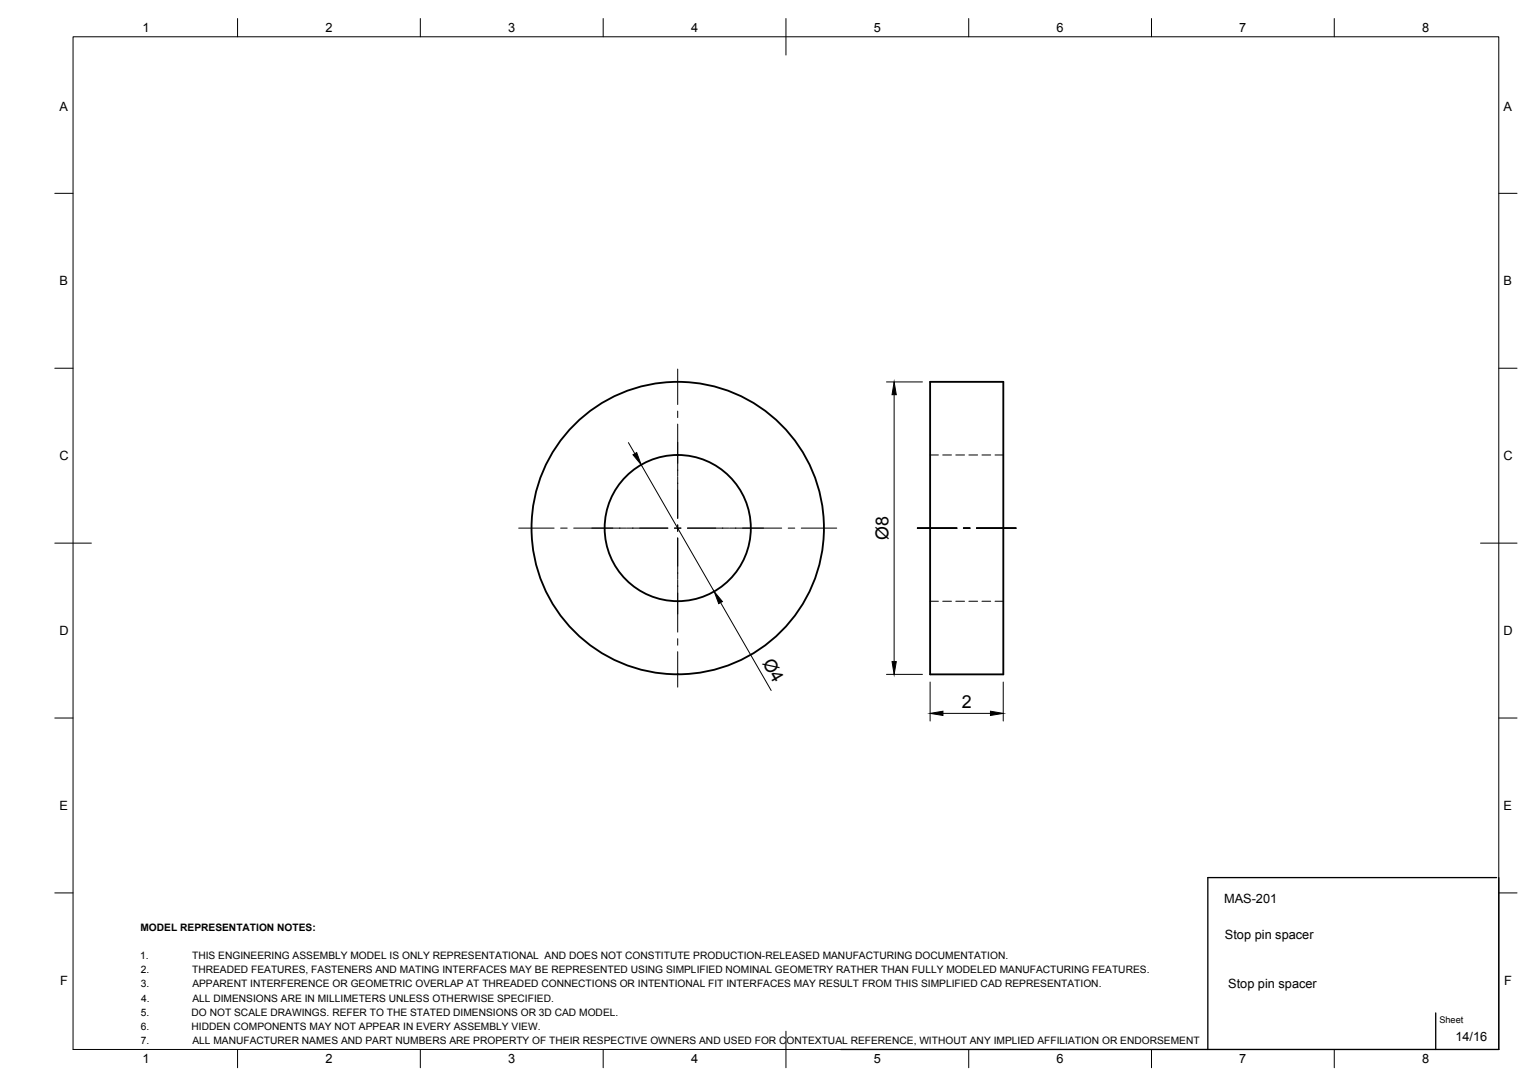
ISO-10303-21;
HEADER;
/* Generated by software containing ST-Developer
 * from STEP Tools, Inc. (www.steptools.com) 
 */

FILE_DESCRIPTION(
/* description */ ('Independent manual two-gate roller-track escapement for nominal30mm d
iameter20mm wide feed rollers. Opposed gates are driven by native capt
ured pin-slot loops with positive curved-slot travel stops at\X\B116de
g. Repeated gate/pin/washer/clip instances, adapted native common bear
ing families, full retaining lips and rotating polymer grip. External 
workpieces, gravity feeder/incline and mount anchors outside assembly.
 No powered-feed compatibility, impact, capacity, safety, force, wear 
or life rating.'),
/* implementation_level */ '2;1');

FILE_NAME(
/* name */ 'Stop pin spacer.step',
/* time_stamp */ '2026-11-08T18:43:23-08:00',
/* author */ (''),
/* organization */ (''),
/* preprocessor_version */ 'ST-DEVELOPER v20.2',
/* originating_system */ 'Autodesk Translation Framework v15.17.0.0',
/* authorisation */ '');

FILE_SCHEMA (('AUTOMOTIVE_DESIGN { 1 0 10303 214 3 1 1 }'));
ENDSEC;

DATA;
#10=MECHANICAL_DESIGN_GEOMETRIC_PRESENTATION_REPRESENTATION('',(#468),#19863);
#430=SHAPE_REPRESENTATION_RELATIONSHIP('SRR','None',#19948,#449);
#449=ADVANCED_BREP_SHAPE_REPRESENTATION('',(#487),#19857);
#468=STYLED_ITEM('',(#20043),#487);
#487=MANIFOLD_SOLID_BREP('Body1',#6437);
#862=LINE('',#15977,#1327);
#863=LINE('',#15983,#1328);
#1327=VECTOR('',#8336,2.);
#1328=VECTOR('',#8343,4.);
#1560=CYLINDRICAL_SURFACE('',#7039,2.);
#1561=CYLINDRICAL_SURFACE('',#7042,4.);
#1676=FACE_BOUND('',#2373,.T.);
#1677=FACE_BOUND('',#2375,.T.);
#1952=FACE_OUTER_BOUND('',#2370,.T.);
#1953=FACE_OUTER_BOUND('',#2371,.T.);
#1954=FACE_OUTER_BOUND('',#2372,.T.);
#1955=FACE_OUTER_BOUND('',#2374,.T.);
#2370=EDGE_LOOP('',(#5457,#5458,#5459,#5460));
#2371=EDGE_LOOP('',(#5461,#5462,#5463,#5464));
#2372=EDGE_LOOP('',(#5465));
#2373=EDGE_LOOP('',(#5466));
#2374=EDGE_LOOP('',(#5467));
#2375=EDGE_LOOP('',(#5468));
#2586=CIRCLE('',#7040,2.);
#2587=CIRCLE('',#7041,2.);
#2588=CIRCLE('',#7043,4.);
#2589=CIRCLE('',#7044,4.);
#3064=VERTEX_POINT('',#15974);
#3065=VERTEX_POINT('',#15976);
#3066=VERTEX_POINT('',#15980);
#3067=VERTEX_POINT('',#15982);
#3887=EDGE_CURVE('',#3064,#3064,#2586,.T.);
#3888=EDGE_CURVE('',#3064,#3065,#862,.T.);
#3889=EDGE_CURVE('',#3065,#3065,#2587,.T.);
#3890=EDGE_CURVE('',#3066,#3066,#2588,.T.);
#3891=EDGE_CURVE('',#3066,#3067,#863,.T.);
#3892=EDGE_CURVE('',#3067,#3067,#2589,.T.);
#5457=ORIENTED_EDGE('',*,*,#3887,.F.);
#5458=ORIENTED_EDGE('',*,*,#3888,.T.);
#5459=ORIENTED_EDGE('',*,*,#3889,.T.);
#5460=ORIENTED_EDGE('',*,*,#3888,.F.);
#5461=ORIENTED_EDGE('',*,*,#3890,.F.);
#5462=ORIENTED_EDGE('',*,*,#3891,.T.);
#5463=ORIENTED_EDGE('',*,*,#3892,.T.);
#5464=ORIENTED_EDGE('',*,*,#3891,.F.);
#5465=ORIENTED_EDGE('',*,*,#3890,.T.);
#5466=ORIENTED_EDGE('',*,*,#3887,.T.);
#5467=ORIENTED_EDGE('',*,*,#3892,.F.);
#5468=ORIENTED_EDGE('',*,*,#3889,.F.);
#6035=PLANE('',#7045);
#6036=PLANE('',#7046);
#6331=ADVANCED_FACE('',(#1952),#1560,.F.);
#6332=ADVANCED_FACE('',(#1953),#1561,.T.);
#6333=ADVANCED_FACE('',(#1954,#1676),#6035,.T.);
#6334=ADVANCED_FACE('',(#1955,#1677),#6036,.F.);
#6437=CLOSED_SHELL('',(#6331,#6332,#6333,#6334));
#7038=AXIS2_PLACEMENT_3D('',#15972,#8330,#8331);
#7039=AXIS2_PLACEMENT_3D('',#15973,#8332,#8333);
#7040=AXIS2_PLACEMENT_3D('',#15975,#8334,#8335);
#7041=AXIS2_PLACEMENT_3D('',#15978,#8337,#8338);
#7042=AXIS2_PLACEMENT_3D('',#15979,#8339,#8340);
#7043=AXIS2_PLACEMENT_3D('',#15981,#8341,#8342);
#7044=AXIS2_PLACEMENT_3D('',#15984,#8344,#8345);
#7045=AXIS2_PLACEMENT_3D('',#15985,#8346,#8347);
#7046=AXIS2_PLACEMENT_3D('',#15986,#8348,#8349);
#8330=DIRECTION('axis',(0.,0.,1.));
#8331=DIRECTION('refdir',(1.,0.,0.));
#8332=DIRECTION('center_axis',(0.,0.,1.));
#8333=DIRECTION('ref_axis',(1.,0.,0.));
#8334=DIRECTION('center_axis',(0.,0.,-1.));
#8335=DIRECTION('ref_axis',(1.,0.,0.));
#8336=DIRECTION('',(0.,0.,-1.));
#8337=DIRECTION('center_axis',(0.,0.,-1.));
#8338=DIRECTION('ref_axis',(1.,0.,0.));
#8339=DIRECTION('center_axis',(0.,0.,1.));
#8340=DIRECTION('ref_axis',(1.,0.,0.));
#8341=DIRECTION('center_axis',(0.,0.,1.));
#8342=DIRECTION('ref_axis',(1.,0.,0.));
#8343=DIRECTION('',(0.,0.,-1.));
#8344=DIRECTION('center_axis',(0.,0.,1.));
#8345=DIRECTION('ref_axis',(1.,0.,0.));
#8346=DIRECTION('center_axis',(0.,0.,1.));
#8347=DIRECTION('ref_axis',(1.,0.,0.));
#8348=DIRECTION('center_axis',(0.,0.,1.));
#8349=DIRECTION('ref_axis',(1.,0.,0.));
#15972=CARTESIAN_POINT('',(0.,0.,0.));
#15973=CARTESIAN_POINT('Origin',(0.,0.,0.));
#15974=CARTESIAN_POINT('',(-2.,-2.44929359829471E-16,2.));
#15975=CARTESIAN_POINT('Origin',(0.,0.,2.));
#15976=CARTESIAN_POINT('',(-2.,-2.44929359829471E-16,0.));
#15977=CARTESIAN_POINT('',(-2.,-2.44929359829471E-16,0.));
#15978=CARTESIAN_POINT('Origin',(0.,0.,0.));
#15979=CARTESIAN_POINT('Origin',(0.,0.,0.));
#15980=CARTESIAN_POINT('',(-4.,-4.89858719658941E-16,2.));
#15981=CARTESIAN_POINT('Origin',(0.,0.,2.));
#15982=CARTESIAN_POINT('',(-4.,-4.89858719658941E-16,0.));
#15983=CARTESIAN_POINT('',(-4.,-4.89858719658941E-16,0.));
#15984=CARTESIAN_POINT('Origin',(0.,0.,0.));
#15985=CARTESIAN_POINT('Origin',(0.,0.,2.));
#15986=CARTESIAN_POINT('Origin',(0.,0.,0.));
#19836=UNCERTAINTY_MEASURE_WITH_UNIT(LENGTH_MEASURE(0.01),#19864,
'DISTANCE_ACCURACY_VALUE',
'Maximum model space distance between geometric entities at asserted c
onnectivities');
#19842=UNCERTAINTY_MEASURE_WITH_UNIT(LENGTH_MEASURE(0.01),#19864,
'DISTANCE_ACCURACY_VALUE',
'Maximum model space distance between geometric entities at asserted c
onnectivities');
#19857=(
GEOMETRIC_REPRESENTATION_CONTEXT(3)
GLOBAL_UNCERTAINTY_ASSIGNED_CONTEXT((#19836))
GLOBAL_UNIT_ASSIGNED_CONTEXT((#19864,#19866,#19867))
REPRESENTATION_CONTEXT('','3D')
);
#19863=(
GEOMETRIC_REPRESENTATION_CONTEXT(3)
GLOBAL_UNCERTAINTY_ASSIGNED_CONTEXT((#19842))
GLOBAL_UNIT_ASSIGNED_CONTEXT((#19864,#19866,#19867))
REPRESENTATION_CONTEXT('','3D')
);
#19864=(
LENGTH_UNIT()
NAMED_UNIT(*)
SI_UNIT(.MILLI.,.METRE.)
);
#19866=(
NAMED_UNIT(*)
PLANE_ANGLE_UNIT()
SI_UNIT($,.RADIAN.)
);
#19867=(
NAMED_UNIT(*)
SI_UNIT($,.STERADIAN.)
SOLID_ANGLE_UNIT()
);
#19882=SHAPE_DEFINITION_REPRESENTATION(#19902,#19948);
#19902=PRODUCT_DEFINITION_SHAPE('',$,#19969);
#19948=SHAPE_REPRESENTATION('',(#7038),#19857);
#19954=PRODUCT_DEFINITION_CONTEXT('part definition',#20016,'design');
#19969=PRODUCT_DEFINITION('Stop pin spacer','Stop pin spacer',#19989,#19954);
#19989=PRODUCT_DEFINITION_FORMATION('',$,#20032);
#20016=APPLICATION_CONTEXT(
'Core Data for Automotive Mechanical Design Process');
#20017=PRODUCT_CONTEXT('part definition',#20016,'mechanical');
#20032=PRODUCT('Stop pin spacer','Stop pin spacer',$,(#20017));
#20043=PRESENTATION_STYLE_ASSIGNMENT((#20050));
#20050=SURFACE_STYLE_USAGE(.BOTH.,#20057);
#20057=SURFACE_SIDE_STYLE('',(#20064));
#20064=SURFACE_STYLE_FILL_AREA(#20071);
#20071=FILL_AREA_STYLE('Light gray',(#20078));
#20078=FILL_AREA_STYLE_COLOUR('Light gray',#20085);
#20085=COLOUR_RGB('Light gray',0.725490196078431,0.752941176470588,0.792156862745098);
ENDSEC;
END-ISO-10303-21;
